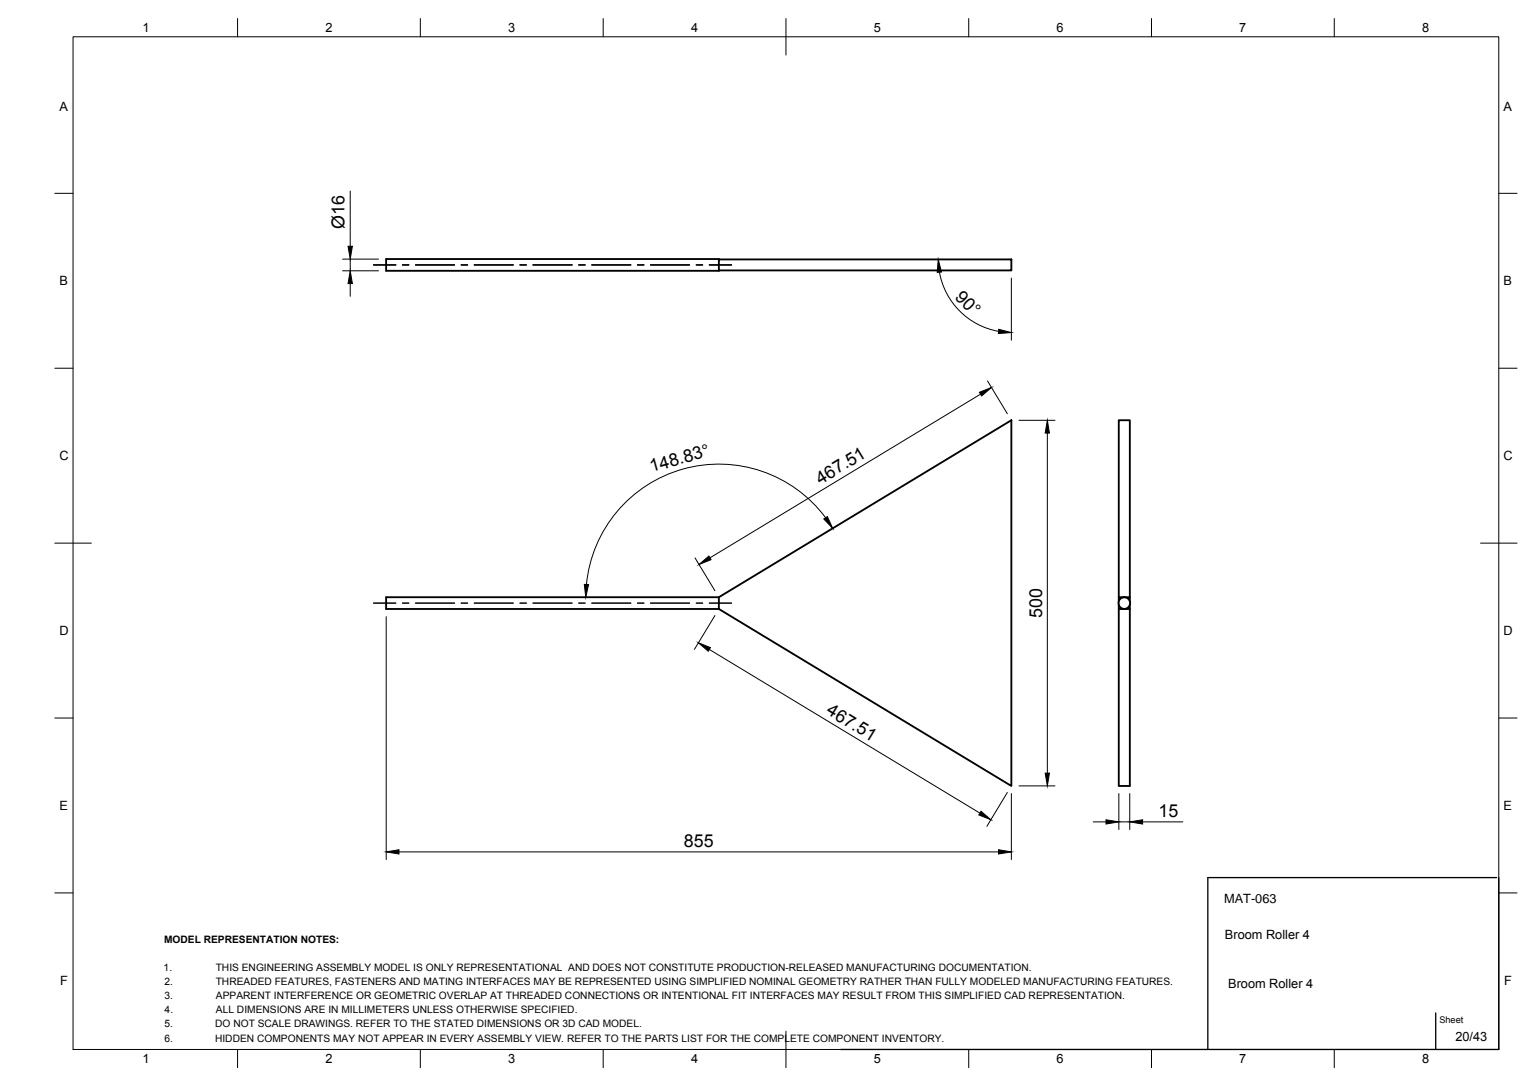
ISO-10303-21;
HEADER;
/* Generated by software containing ST-Developer
 * from STEP Tools, Inc. (www.steptools.com) 
 */

FILE_DESCRIPTION(
/* description */ (''),
/* implementation_level */ '2;1');

FILE_NAME(
/* name */ 'Broom Roller 4.step',
/* time_stamp */ '2026-10-24T09:43:01-07:00',
/* author */ (''),
/* organization */ (''),
/* preprocessor_version */ 'ST-DEVELOPER v20.2',
/* originating_system */ 'Autodesk Translation Framework v15.15.0.0',
/* authorisation */ '');

FILE_SCHEMA (('AUTOMOTIVE_DESIGN { 1 0 10303 214 3 1 1 }'));
ENDSEC;

DATA;
#10=MECHANICAL_DESIGN_GEOMETRIC_PRESENTATION_REPRESENTATION('',(#285),#11112);
#219=SHAPE_REPRESENTATION_RELATIONSHIP('SRR','None',#11243,#252);
#252=ADVANCED_BREP_SHAPE_REPRESENTATION('',(#318),#11088);
#285=STYLED_ITEM('',(#11426),#318);
#318=MANIFOLD_SOLID_BREP('Broom Roller 4',#6022);
#561=PLANE('',#6880);
#562=PLANE('',#6881);
#563=PLANE('',#6882);
#564=PLANE('',#6883);
#565=PLANE('',#6884);
#566=PLANE('',#6885);
#567=PLANE('',#6886);
#568=PLANE('',#6887);
#569=PLANE('',#6888);
#570=PLANE('',#6889);
#571=PLANE('',#6890);
#572=PLANE('',#6891);
#860=FACE_OUTER_BOUND('',#1299,.T.);
#861=FACE_OUTER_BOUND('',#1300,.T.);
#862=FACE_OUTER_BOUND('',#1301,.T.);
#863=FACE_OUTER_BOUND('',#1302,.T.);
#864=FACE_OUTER_BOUND('',#1303,.T.);
#865=FACE_OUTER_BOUND('',#1304,.T.);
#866=FACE_OUTER_BOUND('',#1305,.T.);
#867=FACE_OUTER_BOUND('',#1306,.T.);
#868=FACE_OUTER_BOUND('',#1307,.T.);
#869=FACE_OUTER_BOUND('',#1308,.T.);
#870=FACE_OUTER_BOUND('',#1309,.T.);
#871=FACE_OUTER_BOUND('',#1310,.T.);
#872=FACE_OUTER_BOUND('',#1311,.T.);
#1299=EDGE_LOOP('',(#4745,#4746,#4747,#4748,#4749,#4750,#4751,#4752,#4753,
#4754));
#1300=EDGE_LOOP('',(#4755));
#1301=EDGE_LOOP('',(#4756,#4757,#4758));
#1302=EDGE_LOOP('',(#4759,#4760,#4761));
#1303=EDGE_LOOP('',(#4762,#4763,#4764));
#1304=EDGE_LOOP('',(#4765,#4766));
#1305=EDGE_LOOP('',(#4767,#4768,#4769));
#1306=EDGE_LOOP('',(#4770,#4771,#4772));
#1307=EDGE_LOOP('',(#4773,#4774,#4775,#4776,#4777,#4778));
#1308=EDGE_LOOP('',(#4779,#4780,#4781,#4782,#4783));
#1309=EDGE_LOOP('',(#4784,#4785,#4786,#4787,#4788,#4789));
#1310=EDGE_LOOP('',(#4790,#4791,#4792,#4793,#4794));
#1311=EDGE_LOOP('',(#4795,#4796,#4797,#4798));
#1692=LINE('',#10184,#2051);
#1693=LINE('',#10193,#2052);
#1694=LINE('',#10196,#2053);
#1695=LINE('',#10197,#2054);
#1696=LINE('',#10200,#2055);
#1697=LINE('',#10201,#2056);
#1698=LINE('',#10203,#2057);
#1699=LINE('',#10206,#2058);
#1700=LINE('',#10207,#2059);
#1701=LINE('',#10210,#2060);
#1702=LINE('',#10211,#2061);
#1703=LINE('',#10214,#2062);
#1704=LINE('',#10216,#2063);
#1705=LINE('',#10217,#2064);
#1706=LINE('',#10220,#2065);
#1707=LINE('',#10221,#2066);
#1708=LINE('',#10224,#2067);
#1709=LINE('',#10225,#2068);
#1710=LINE('',#10227,#2069);
#2051=VECTOR('',#8332,0.00799999974118007);
#2052=VECTOR('',#8345,0.01);
#2053=VECTOR('',#8348,0.01);
#2054=VECTOR('',#8349,0.01);
#2055=VECTOR('',#8352,0.01);
#2056=VECTOR('',#8353,0.01);
#2057=VECTOR('',#8356,0.01);
#2058=VECTOR('',#8359,0.01);
#2059=VECTOR('',#8360,0.01);
#2060=VECTOR('',#8363,0.01);
#2061=VECTOR('',#8364,0.01);
#2062=VECTOR('',#8367,0.01);
#2063=VECTOR('',#8368,0.01);
#2064=VECTOR('',#8369,0.01);
#2065=VECTOR('',#8372,0.01);
#2066=VECTOR('',#8373,0.01);
#2067=VECTOR('',#8376,0.01);
#2068=VECTOR('',#8377,0.01);
#2069=VECTOR('',#8380,0.01);
#2538=CIRCLE('',#6872,0.00799999974118007);
#2539=CIRCLE('',#6873,0.00799999974118007);
#2540=CIRCLE('',#6874,0.00799999974118007);
#2541=CIRCLE('',#6875,0.00799999974118007);
#2542=CIRCLE('',#6876,0.00799999974118007);
#2543=CIRCLE('',#6877,0.00799999974118007);
#2544=CIRCLE('',#6878,0.00799999974118007);
#2545=CIRCLE('',#6879,0.00799999974118007);
#2932=VERTEX_POINT('',#10174);
#2933=VERTEX_POINT('',#10175);
#2934=VERTEX_POINT('',#10177);
#2935=VERTEX_POINT('',#10179);
#2936=VERTEX_POINT('',#10181);
#2937=VERTEX_POINT('',#10183);
#2938=VERTEX_POINT('',#10186);
#2939=VERTEX_POINT('',#10188);
#2940=VERTEX_POINT('',#10195);
#2941=VERTEX_POINT('',#10199);
#2942=VERTEX_POINT('',#10205);
#2943=VERTEX_POINT('',#10209);
#2944=VERTEX_POINT('',#10213);
#2945=VERTEX_POINT('',#10215);
#2946=VERTEX_POINT('',#10219);
#2947=VERTEX_POINT('',#10223);
#3576=EDGE_CURVE('',#2932,#2933,#2538,.F.);
#3577=EDGE_CURVE('',#2933,#2934,#2539,.F.);
#3578=EDGE_CURVE('',#2934,#2935,#2540,.F.);
#3579=EDGE_CURVE('',#2935,#2936,#2541,.F.);
#3580=EDGE_CURVE('',#2936,#2937,#1692,.T.);
#3581=EDGE_CURVE('',#2937,#2937,#2542,.T.);
#3582=EDGE_CURVE('',#2936,#2938,#2543,.F.);
#3583=EDGE_CURVE('',#2938,#2939,#2544,.F.);
#3584=EDGE_CURVE('',#2939,#2932,#2545,.F.);
#3585=EDGE_CURVE('',#2935,#2938,#1693,.T.);
#3586=EDGE_CURVE('',#2940,#2939,#1694,.T.);
#3587=EDGE_CURVE('',#2938,#2940,#1695,.T.);
#3588=EDGE_CURVE('',#2941,#2932,#1696,.T.);
#3589=EDGE_CURVE('',#2939,#2941,#1697,.T.);
#3590=EDGE_CURVE('',#2932,#2933,#1698,.T.);
#3591=EDGE_CURVE('',#2942,#2934,#1699,.T.);
#3592=EDGE_CURVE('',#2933,#2942,#1700,.T.);
#3593=EDGE_CURVE('',#2943,#2935,#1701,.T.);
#3594=EDGE_CURVE('',#2934,#2943,#1702,.T.);
#3595=EDGE_CURVE('',#2944,#2943,#1703,.T.);
#3596=EDGE_CURVE('',#2945,#2944,#1704,.T.);
#3597=EDGE_CURVE('',#2940,#2945,#1705,.T.);
#3598=EDGE_CURVE('',#2946,#2945,#1706,.T.);
#3599=EDGE_CURVE('',#2941,#2946,#1707,.T.);
#3600=EDGE_CURVE('',#2946,#2947,#1708,.T.);
#3601=EDGE_CURVE('',#2947,#2942,#1709,.T.);
#3602=EDGE_CURVE('',#2947,#2944,#1710,.T.);
#4745=ORIENTED_EDGE('',*,*,#3576,.T.);
#4746=ORIENTED_EDGE('',*,*,#3577,.T.);
#4747=ORIENTED_EDGE('',*,*,#3578,.T.);
#4748=ORIENTED_EDGE('',*,*,#3579,.T.);
#4749=ORIENTED_EDGE('',*,*,#3580,.T.);
#4750=ORIENTED_EDGE('',*,*,#3581,.T.);
#4751=ORIENTED_EDGE('',*,*,#3580,.F.);
#4752=ORIENTED_EDGE('',*,*,#3582,.T.);
#4753=ORIENTED_EDGE('',*,*,#3583,.T.);
#4754=ORIENTED_EDGE('',*,*,#3584,.T.);
#4755=ORIENTED_EDGE('',*,*,#3581,.F.);
#4756=ORIENTED_EDGE('',*,*,#3585,.T.);
#4757=ORIENTED_EDGE('',*,*,#3582,.F.);
#4758=ORIENTED_EDGE('',*,*,#3579,.F.);
#4759=ORIENTED_EDGE('',*,*,#3586,.T.);
#4760=ORIENTED_EDGE('',*,*,#3583,.F.);
#4761=ORIENTED_EDGE('',*,*,#3587,.T.);
#4762=ORIENTED_EDGE('',*,*,#3588,.T.);
#4763=ORIENTED_EDGE('',*,*,#3584,.F.);
#4764=ORIENTED_EDGE('',*,*,#3589,.T.);
#4765=ORIENTED_EDGE('',*,*,#3590,.T.);
#4766=ORIENTED_EDGE('',*,*,#3576,.F.);
#4767=ORIENTED_EDGE('',*,*,#3591,.T.);
#4768=ORIENTED_EDGE('',*,*,#3577,.F.);
#4769=ORIENTED_EDGE('',*,*,#3592,.T.);
#4770=ORIENTED_EDGE('',*,*,#3593,.T.);
#4771=ORIENTED_EDGE('',*,*,#3578,.F.);
#4772=ORIENTED_EDGE('',*,*,#3594,.T.);
#4773=ORIENTED_EDGE('',*,*,#3595,.F.);
#4774=ORIENTED_EDGE('',*,*,#3596,.F.);
#4775=ORIENTED_EDGE('',*,*,#3597,.F.);
#4776=ORIENTED_EDGE('',*,*,#3587,.F.);
#4777=ORIENTED_EDGE('',*,*,#3585,.F.);
#4778=ORIENTED_EDGE('',*,*,#3593,.F.);
#4779=ORIENTED_EDGE('',*,*,#3586,.F.);
#4780=ORIENTED_EDGE('',*,*,#3597,.T.);
#4781=ORIENTED_EDGE('',*,*,#3598,.F.);
#4782=ORIENTED_EDGE('',*,*,#3599,.F.);
#4783=ORIENTED_EDGE('',*,*,#3589,.F.);
#4784=ORIENTED_EDGE('',*,*,#3600,.T.);
#4785=ORIENTED_EDGE('',*,*,#3601,.T.);
#4786=ORIENTED_EDGE('',*,*,#3592,.F.);
#4787=ORIENTED_EDGE('',*,*,#3590,.F.);
#4788=ORIENTED_EDGE('',*,*,#3588,.F.);
#4789=ORIENTED_EDGE('',*,*,#3599,.T.);
#4790=ORIENTED_EDGE('',*,*,#3595,.T.);
#4791=ORIENTED_EDGE('',*,*,#3594,.F.);
#4792=ORIENTED_EDGE('',*,*,#3591,.F.);
#4793=ORIENTED_EDGE('',*,*,#3601,.F.);
#4794=ORIENTED_EDGE('',*,*,#3602,.T.);
#4795=ORIENTED_EDGE('',*,*,#3598,.T.);
#4796=ORIENTED_EDGE('',*,*,#3596,.T.);
#4797=ORIENTED_EDGE('',*,*,#3602,.F.);
#4798=ORIENTED_EDGE('',*,*,#3600,.F.);
#5573=CYLINDRICAL_SURFACE('',#6871,0.00799999974118007);
#5833=ADVANCED_FACE('',(#860),#5573,.T.);
#5834=ADVANCED_FACE('',(#861),#561,.F.);
#5835=ADVANCED_FACE('',(#862),#562,.T.);
#5836=ADVANCED_FACE('',(#863),#563,.T.);
#5837=ADVANCED_FACE('',(#864),#564,.T.);
#5838=ADVANCED_FACE('',(#865),#565,.T.);
#5839=ADVANCED_FACE('',(#866),#566,.T.);
#5840=ADVANCED_FACE('',(#867),#567,.T.);
#5841=ADVANCED_FACE('',(#868),#568,.F.);
#5842=ADVANCED_FACE('',(#869),#569,.F.);
#5843=ADVANCED_FACE('',(#870),#570,.T.);
#5844=ADVANCED_FACE('',(#871),#571,.T.);
#5845=ADVANCED_FACE('',(#872),#572,.F.);
#6022=CLOSED_SHELL('',(#5833,#5834,#5835,#5836,#5837,#5838,#5839,#5840,
#5841,#5842,#5843,#5844,#5845));
#6870=AXIS2_PLACEMENT_3D('',#10172,#8320,#8321);
#6871=AXIS2_PLACEMENT_3D('',#10173,#8322,#8323);
#6872=AXIS2_PLACEMENT_3D('',#10176,#8324,#8325);
#6873=AXIS2_PLACEMENT_3D('',#10178,#8326,#8327);
#6874=AXIS2_PLACEMENT_3D('',#10180,#8328,#8329);
#6875=AXIS2_PLACEMENT_3D('',#10182,#8330,#8331);
#6876=AXIS2_PLACEMENT_3D('',#10185,#8333,#8334);
#6877=AXIS2_PLACEMENT_3D('',#10187,#8335,#8336);
#6878=AXIS2_PLACEMENT_3D('',#10189,#8337,#8338);
#6879=AXIS2_PLACEMENT_3D('',#10190,#8339,#8340);
#6880=AXIS2_PLACEMENT_3D('',#10191,#8341,#8342);
#6881=AXIS2_PLACEMENT_3D('',#10192,#8343,#8344);
#6882=AXIS2_PLACEMENT_3D('',#10194,#8346,#8347);
#6883=AXIS2_PLACEMENT_3D('',#10198,#8350,#8351);
#6884=AXIS2_PLACEMENT_3D('',#10202,#8354,#8355);
#6885=AXIS2_PLACEMENT_3D('',#10204,#8357,#8358);
#6886=AXIS2_PLACEMENT_3D('',#10208,#8361,#8362);
#6887=AXIS2_PLACEMENT_3D('',#10212,#8365,#8366);
#6888=AXIS2_PLACEMENT_3D('',#10218,#8370,#8371);
#6889=AXIS2_PLACEMENT_3D('',#10222,#8374,#8375);
#6890=AXIS2_PLACEMENT_3D('',#10226,#8378,#8379);
#6891=AXIS2_PLACEMENT_3D('',#10228,#8381,#8382);
#8320=DIRECTION('axis',(0.,0.,1.));
#8321=DIRECTION('refdir',(1.,0.,0.));
#8322=DIRECTION('center_axis',(0.,0.604097518614064,0.796910401490865));
#8323=DIRECTION('ref_axis',(0.,-0.796910401490865,0.604097518614064));
#8324=DIRECTION('center_axis',(0.,0.604097518614064,0.796910401490865));
#8325=DIRECTION('ref_axis',(0.,-0.796910401490865,0.604097518614064));
#8326=DIRECTION('center_axis',(0.,0.604097518614064,0.796910401490865));
#8327=DIRECTION('ref_axis',(0.,-0.796910401490865,0.604097518614064));
#8328=DIRECTION('center_axis',(0.,0.604097518614064,0.796910401490865));
#8329=DIRECTION('ref_axis',(0.,-0.796910401490865,0.604097518614064));
#8330=DIRECTION('center_axis',(0.,0.604097518614064,0.796910401490865));
#8331=DIRECTION('ref_axis',(0.,-0.796910401490865,0.604097518614064));
#8332=DIRECTION('',(0.,-0.604097518614064,-0.796910401490865));
#8333=DIRECTION('center_axis',(0.,0.604097518614064,0.796910401490865));
#8334=DIRECTION('ref_axis',(0.,-0.796910401490865,0.604097518614064));
#8335=DIRECTION('center_axis',(0.,0.604097518614064,0.796910401490865));
#8336=DIRECTION('ref_axis',(0.,-0.796910401490865,0.604097518614064));
#8337=DIRECTION('center_axis',(0.,0.604097518614064,0.796910401490865));
#8338=DIRECTION('ref_axis',(0.,-0.796910401490865,0.604097518614064));
#8339=DIRECTION('center_axis',(0.,0.604097518614064,0.796910401490865));
#8340=DIRECTION('ref_axis',(0.,-0.796910401490865,0.604097518614064));
#8341=DIRECTION('center_axis',(1.76011166144385E-16,0.604097524343638,0.796910397147564));
#8342=DIRECTION('ref_axis',(-5.69382634799286E-34,-0.796910397147564,0.604097524343638));
#8343=DIRECTION('center_axis',(-2.4695605328884E-15,0.604097388004457,0.796910500499393));
#8344=DIRECTION('ref_axis',(-2.15217716924996E-31,-0.796910500499393,0.604097388004457));
#8345=DIRECTION('',(1.,0.,0.));
#8346=DIRECTION('center_axis',(5.0257917292328E-15,-0.604097535980688,-0.796910388326104));
#8347=DIRECTION('ref_axis',(3.96880149093465E-31,0.796910388326104,-0.604097535980688));
#8348=DIRECTION('',(9.06795873383563E-9,-0.796910391640021,0.60409753160905));
#8349=DIRECTION('',(1.,0.,0.));
#8350=DIRECTION('center_axis',(-1.3539365332793E-15,-0.604097535980685,
-0.796910388326106));
#8351=DIRECTION('ref_axis',(-3.09014762786369E-33,0.796910388326106,-0.604097535980685));
#8352=DIRECTION('',(-1.,0.,0.));
#8353=DIRECTION('',(9.06765857867901E-9,-0.796910391640318,0.60409753160866));
#8354=DIRECTION('center_axis',(1.30898403527359E-14,0.604097388004449,0.796910500499399));
#8355=DIRECTION('ref_axis',(7.65782089424487E-31,-0.796910500499399,0.604097388004449));
#8356=DIRECTION('',(-1.,1.78664147484789E-13,0.));
#8357=DIRECTION('center_axis',(-1.36705691295974E-15,-0.604097535980685,
-0.796910388326106));
#8358=DIRECTION('ref_axis',(-4.01110836398031E-32,0.796910388326106,-0.604097535980685));
#8359=DIRECTION('',(9.06797358508429E-9,0.796910391640005,-0.604097531609072));
#8360=DIRECTION('',(-1.,0.,0.));
#8361=DIRECTION('center_axis',(2.86322345620586E-16,-0.604097535980689,
-0.796910388326103));
#8362=DIRECTION('ref_axis',(4.76719382107084E-33,0.796910388326103,-0.604097535980689));
#8363=DIRECTION('',(1.,0.,0.));
#8364=DIRECTION('',(9.06768872847231E-9,0.796910391640293,-0.604097531608692));
#8365=DIRECTION('center_axis',(1.49607962990053E-17,-0.796910402395455,
0.604097517420751));
#8366=DIRECTION('ref_axis',(6.62628247037524E-34,-0.604097517420751,-0.796910402395455));
#8367=DIRECTION('',(0.517637881323564,-0.516865717224615,-0.68183638372907));
#8368=DIRECTION('',(-1.,0.,0.));
#8369=DIRECTION('',(0.517637881323564,0.516865717224616,0.68183638372907));
#8370=DIRECTION('center_axis',(-0.855599803540681,0.312703760192046,0.412511011420185));
#8371=DIRECTION('ref_axis',(0.434290367983341,3.1478940293141E-16,0.900772932695524));
#8372=DIRECTION('',(-6.812600991711E-9,0.796910393860769,-0.604097528679495));
#8373=DIRECTION('',(0.517637881323564,0.516865717224607,0.681836383729077));
#8374=DIRECTION('center_axis',(2.02339551431575E-18,-0.796910402395456,
0.60409751742075));
#8375=DIRECTION('ref_axis',(2.11465894662532E-34,-0.60409751742075,-0.796910402395456));
#8376=DIRECTION('',(-1.,0.,0.));
#8377=DIRECTION('',(0.517637881323564,-0.516865717224604,-0.681836383729078));
#8378=DIRECTION('center_axis',(-0.855599803540681,-0.312703760192046,-0.412511011420185));
#8379=DIRECTION('ref_axis',(-0.434290367983341,3.1478940293141E-16,0.900772932695524));
#8380=DIRECTION('',(6.812600991711E-9,0.796910393860769,-0.604097528679495));
#8381=DIRECTION('center_axis',(-4.61706709228339E-17,-0.604097528679492,
-0.796910393860772));
#8382=DIRECTION('ref_axis',(-3.71158212193438E-33,0.796910393860772,-0.604097528679492));
#10172=CARTESIAN_POINT('',(0.,0.,0.));
#10173=CARTESIAN_POINT('Origin',(0.,0.377184388,1.135860968));
#10174=CARTESIAN_POINT('',(0.00278388195593357,0.64607193114008,1.50298593209025));
#10175=CARTESIAN_POINT('',(-0.00278388195593361,0.64607193114008,1.50298593209025));
#10176=CARTESIAN_POINT('Origin',(0.,0.652048759141067,1.4984552009048));
#10177=CARTESIAN_POINT('',(-0.00799999980513634,0.652048759131474,1.49845520070589));
#10178=CARTESIAN_POINT('Origin',(0.,0.652048759141067,1.4984552009048));
#10179=CARTESIAN_POINT('',(-0.00278388142421084,0.658025587080488,1.49392446925429));
#10180=CARTESIAN_POINT('Origin',(0.,0.652048759141067,1.4984552009048));
#10181=CARTESIAN_POINT('',(-9.79717407621583E-19,0.658424042146736,1.49362242091224));
#10182=CARTESIAN_POINT('Origin',(0.,0.652048759141067,1.4984552009048));
#10183=CARTESIAN_POINT('',(-9.79717407621583E-19,0.383559671011319,1.13102818801489));
#10184=CARTESIAN_POINT('',(-9.79717407621583E-19,0.383559671005671,1.13102818800744));
#10185=CARTESIAN_POINT('Origin',(0.,0.377184388005651,1.13586096800745));
#10186=CARTESIAN_POINT('',(0.00278388142421076,0.658025587080488,1.49392446925429));
#10187=CARTESIAN_POINT('Origin',(0.,0.652048759141067,1.4984552009048));
#10188=CARTESIAN_POINT('',(0.00799999980513743,0.652048759130905,1.49845520070633));
#10189=CARTESIAN_POINT('Origin',(0.,0.652048759141067,1.4984552009048));
#10190=CARTESIAN_POINT('Origin',(0.,0.652048759141067,1.4984552009048));
#10191=CARTESIAN_POINT('Origin',(-1.99493199737333E-19,0.3771843885,1.1358609685));
#10192=CARTESIAN_POINT('Origin',(-2.16840434497101E-21,0.658224814634137,
1.49377344464617));
#10193=CARTESIAN_POINT('',(-0.00278388206047001,0.658025587,1.493924469));
#10194=CARTESIAN_POINT('Origin',(0.0053919408556245,0.655037172984959,1.49618983480451));
#10195=CARTESIAN_POINT('',(0.00799999981595462,0.658025587031806,1.49392446904196));
#10196=CARTESIAN_POINT('',(0.00799999983151832,0.658025587061577,1.49392446908123));
#10197=CARTESIAN_POINT('',(0.00278388206047,0.658025587,1.493924469));
#10198=CARTESIAN_POINT('Origin',(0.0053919408556245,0.64906034501504,1.50072056619548));
#10199=CARTESIAN_POINT('',(0.00799999989834483,0.64607193101772,1.50298593202338));
#10200=CARTESIAN_POINT('',(0.00800000000000001,0.646071930999999,1.502985932));
#10201=CARTESIAN_POINT('',(0.00799999983866159,0.65204875900126,1.49845520053531));
#10202=CARTESIAN_POINT('Origin',(-2.16840434497101E-21,0.645872703365862,
1.50313695635384));
#10203=CARTESIAN_POINT('',(0.00278388206047,0.646071930999999,1.502985932));
#10204=CARTESIAN_POINT('Origin',(-0.00539194085562444,0.64906034501504,
1.50072056619548));
#10205=CARTESIAN_POINT('',(-0.00799999989827039,0.646071931017694,1.50298593202334));
#10206=CARTESIAN_POINT('',(-0.00799999990666903,0.64607193103411,1.502985932045));
#10207=CARTESIAN_POINT('',(-0.00278388206047,0.646071930999999,1.502985932));
#10208=CARTESIAN_POINT('Origin',(-0.00539194085562444,0.655037172984959,
1.49618983480451));
#10209=CARTESIAN_POINT('',(-0.00799999981595463,0.658025587031806,1.49392446904196));
#10210=CARTESIAN_POINT('',(-0.00799999999999999,0.658025587,1.493924469));
#10211=CARTESIAN_POINT('',(-0.00799999989952599,0.652048759062608,1.49845520061504));
#10212=CARTESIAN_POINT('Origin',(-8.88178419700125E-18,0.778845090499999,
1.6533065495));
#10213=CARTESIAN_POINT('',(-0.249999999783566,0.899664593989047,1.81268862998555));
#10214=CARTESIAN_POINT('',(-0.249999999796965,0.899664593910672,1.81268862988216));
#10215=CARTESIAN_POINT('',(0.249999999783566,0.899664593989047,1.81268862998555));
#10216=CARTESIAN_POINT('',(0.249999999800629,0.899664593999999,1.81268863));
#10217=CARTESIAN_POINT('',(0.00799999985480845,0.658025587084829,1.49392446911191));
#10218=CARTESIAN_POINT('Origin',(0.129,0.772868262499999,1.65783728125));
#10219=CARTESIAN_POINT('',(0.249999999885983,0.88771093798903,1.82175009298553));
#10220=CARTESIAN_POINT('',(0.2499999998105,0.887710938334042,1.82175009274678));
#10221=CARTESIAN_POINT('',(0.00800000016977363,0.646071931296823,1.50298593239156));
#10222=CARTESIAN_POINT('Origin',(-8.88178419700125E-18,0.7668914345,1.6623680125));
#10223=CARTESIAN_POINT('',(-0.24999999988596,0.88771093798902,1.82175009298552));
#10224=CARTESIAN_POINT('',(0.249999999800629,0.887710938,1.821750093));
#10225=CARTESIAN_POINT('',(-0.24999999988113,0.887710937892202,1.8217500928578));
#10226=CARTESIAN_POINT('Origin',(-0.129,0.772868262499999,1.65783728125));
#10227=CARTESIAN_POINT('',(-0.2499999998105,0.887710938334042,1.82175009274678));
#10228=CARTESIAN_POINT('Origin',(-8.88178419700125E-18,0.893687766,1.8172193615));
#11049=UNCERTAINTY_MEASURE_WITH_UNIT(LENGTH_MEASURE(1.E-5),#11113,
'DISTANCE_ACCURACY_VALUE',
'Maximum model space distance between geometric entities at asserted c
onnectivities');
#11073=UNCERTAINTY_MEASURE_WITH_UNIT(LENGTH_MEASURE(1.E-5),#11113,
'DISTANCE_ACCURACY_VALUE',
'Maximum model space distance between geometric entities at asserted c
onnectivities');
#11088=(
GEOMETRIC_REPRESENTATION_CONTEXT(3)
GLOBAL_UNCERTAINTY_ASSIGNED_CONTEXT((#11049))
GLOBAL_UNIT_ASSIGNED_CONTEXT((#11113,#11114,#11115))
REPRESENTATION_CONTEXT('','3D')
);
#11112=(
GEOMETRIC_REPRESENTATION_CONTEXT(3)
GLOBAL_UNCERTAINTY_ASSIGNED_CONTEXT((#11073))
GLOBAL_UNIT_ASSIGNED_CONTEXT((#11113,#11114,#11115))
REPRESENTATION_CONTEXT('','3D')
);
#11113=(
LENGTH_UNIT()
NAMED_UNIT(*)
SI_UNIT($,.METRE.)
);
#11114=(
NAMED_UNIT(*)
PLANE_ANGLE_UNIT()
SI_UNIT($,.RADIAN.)
);
#11115=(
NAMED_UNIT(*)
SI_UNIT($,.STERADIAN.)
SOLID_ANGLE_UNIT()
);
#11130=SHAPE_DEFINITION_REPRESENTATION(#11168,#11243);
#11168=PRODUCT_DEFINITION_SHAPE('',$,#11282);
#11243=SHAPE_REPRESENTATION('',(#6870),#11088);
#11267=PRODUCT_DEFINITION_CONTEXT('part definition',#11383,'design');
#11282=PRODUCT_DEFINITION('Broom Roller 4','Broom Roller 4',#11320,#11267);
#11320=PRODUCT_DEFINITION_FORMATION('',$,#11399);
#11383=APPLICATION_CONTEXT(
'Core Data for Automotive Mechanical Design Process');
#11384=PRODUCT_CONTEXT('part definition',#11383,'mechanical');
#11399=PRODUCT('Broom Roller 4','Broom Roller 4',
'broom_and_roller__ DE     5607',(#11384));
#11426=PRESENTATION_STYLE_ASSIGNMENT((#11430));
#11430=SURFACE_STYLE_USAGE(.BOTH.,#11434);
#11434=SURFACE_SIDE_STYLE('',(#11438));
#11438=SURFACE_STYLE_FILL_AREA(#11442);
#11442=FILL_AREA_STYLE('Opaque(202,209,238)',(#11446));
#11446=FILL_AREA_STYLE_COLOUR('Opaque(202,209,238)',#11450);
#11450=COLOUR_RGB('Opaque(202,209,238)',0.792156862745098,0.819607843137255,
0.933333333333333);
ENDSEC;
END-ISO-10303-21;
